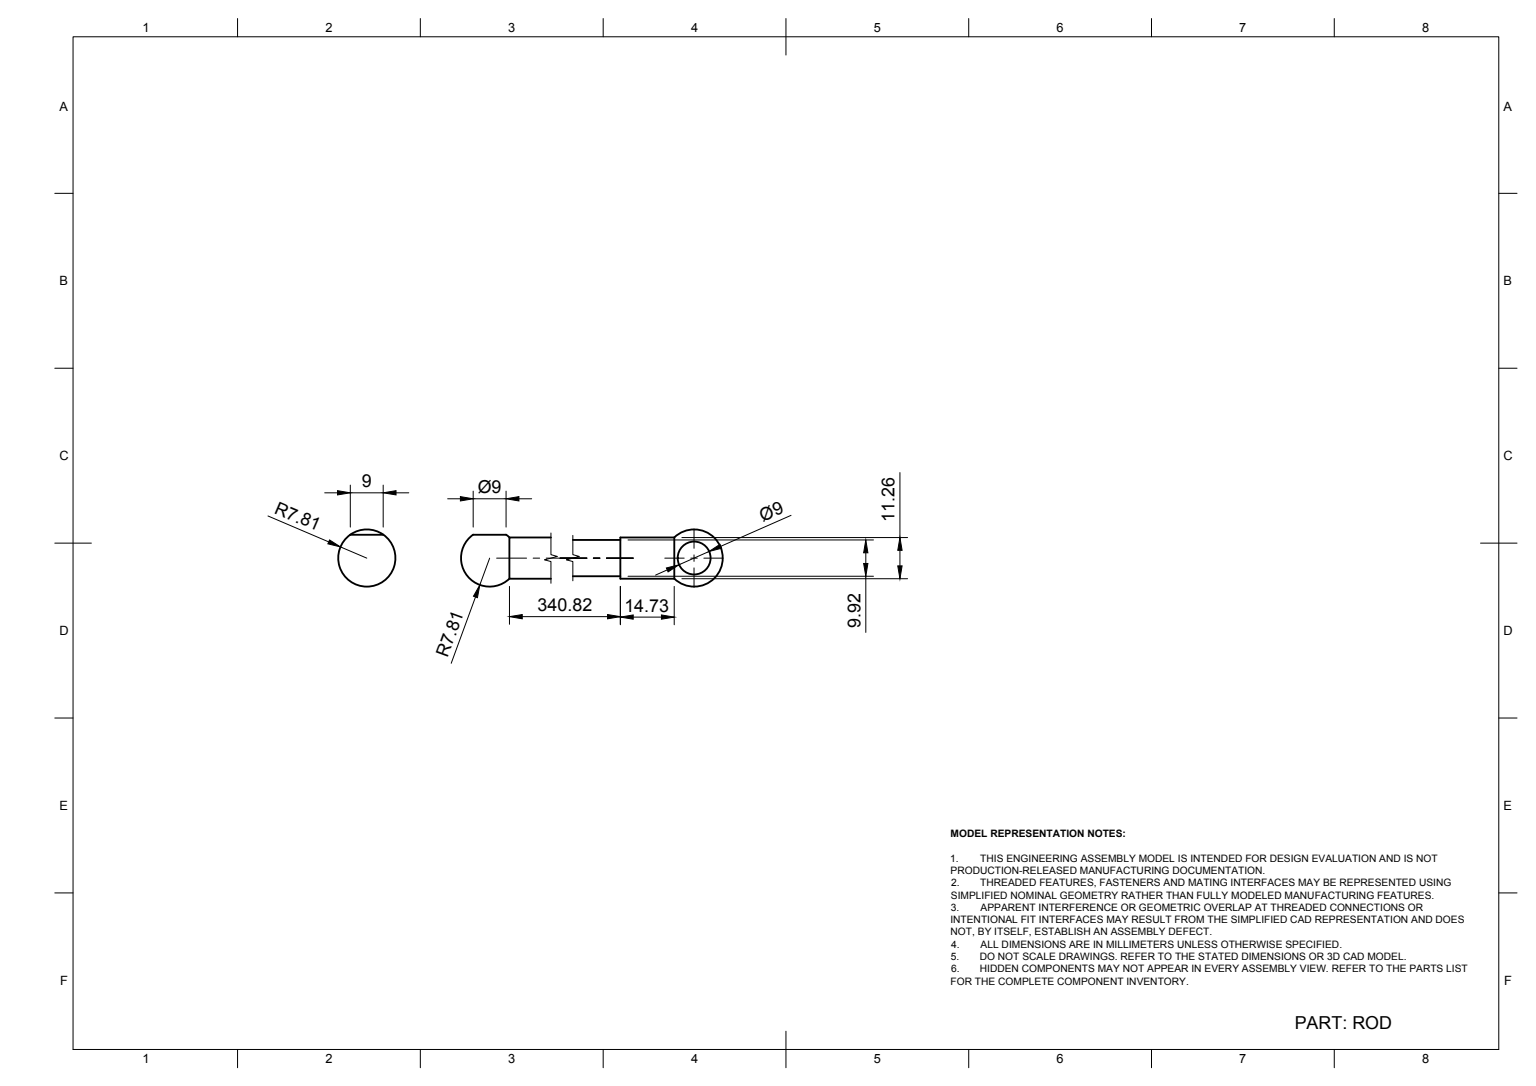
ISO-10303-21;
HEADER;
/* Generated by software containing ST-Developer
 * from STEP Tools, Inc. (www.steptools.com) 
 */

FILE_DESCRIPTION(
/* description */ (''),
/* implementation_level */ '2;1');

FILE_NAME(
/* name */ 'Rod.step',
/* time_stamp */ '2026-10-04T16:49:01-07:00',
/* author */ (''),
/* organization */ (''),
/* preprocessor_version */ 'ST-DEVELOPER v20.2',
/* originating_system */ 'Autodesk Translation Framework v15.15.0.0',
/* authorisation */ '');

FILE_SCHEMA (('AUTOMOTIVE_DESIGN { 1 0 10303 214 3 1 1 }'));
ENDSEC;

DATA;
#10=MECHANICAL_DESIGN_GEOMETRIC_PRESENTATION_REPRESENTATION('',(#87,#88),#51553);
#43=SPHERICAL_SURFACE('',#4646,7.81234603703673);
#44=SPHERICAL_SURFACE('',#4651,7.81234603703673);
#71=SHAPE_REPRESENTATION_RELATIONSHIP('SRR','None',#51592,#79);
#79=ADVANCED_BREP_SHAPE_REPRESENTATION('',(#96,#97),#51552);
#87=STYLED_ITEM('',(#51634),#96);
#88=STYLED_ITEM('',(#51634),#97);
#96=MANIFOLD_SOLID_BREP('Body1',#4266);
#97=MANIFOLD_SOLID_BREP('Body2',#4267);
#116=FACE_BOUND('',#579,.T.);
#117=FACE_BOUND('',#583,.T.);
#118=FACE_BOUND('',#586,.T.);
#119=FACE_BOUND('',#591,.T.);
#175=PLANE('',#4632);
#176=PLANE('',#4637);
#177=PLANE('',#4639);
#178=PLANE('',#4658);
#179=PLANE('',#4661);
#180=PLANE('',#4662);
#362=FACE_OUTER_BOUND('',#575,.T.);
#363=FACE_OUTER_BOUND('',#576,.T.);
#364=FACE_OUTER_BOUND('',#577,.T.);
#365=FACE_OUTER_BOUND('',#578,.T.);
#366=FACE_OUTER_BOUND('',#580,.T.);
#367=FACE_OUTER_BOUND('',#581,.T.);
#368=FACE_OUTER_BOUND('',#582,.T.);
#369=FACE_OUTER_BOUND('',#584,.T.);
#370=FACE_OUTER_BOUND('',#585,.T.);
#371=FACE_OUTER_BOUND('',#587,.T.);
#372=FACE_OUTER_BOUND('',#588,.T.);
#373=FACE_OUTER_BOUND('',#589,.T.);
#374=FACE_OUTER_BOUND('',#590,.T.);
#375=FACE_OUTER_BOUND('',#592,.T.);
#575=EDGE_LOOP('',(#3895,#3896,#3897,#3898,#3899));
#576=EDGE_LOOP('',(#3900,#3901,#3902,#3903,#3904,#3905,#3906));
#577=EDGE_LOOP('',(#3907,#3908));
#578=EDGE_LOOP('',(#3909));
#579=EDGE_LOOP('',(#3910));
#580=EDGE_LOOP('',(#3911,#3912,#3913,#3914,#3915,#3916,#3917,#3918));
#581=EDGE_LOOP('',(#3919,#3920,#3921,#3922,#3923));
#582=EDGE_LOOP('',(#3924,#3925,#3926,#3927));
#583=EDGE_LOOP('',(#3928));
#584=EDGE_LOOP('',(#3929,#3930,#3931,#3932));
#585=EDGE_LOOP('',(#3933,#3934,#3935,#3936));
#586=EDGE_LOOP('',(#3937));
#587=EDGE_LOOP('',(#3938,#3939,#3940,#3941,#3942));
#588=EDGE_LOOP('',(#3943));
#589=EDGE_LOOP('',(#3944,#3945,#3946,#3947));
#590=EDGE_LOOP('',(#3948));
#591=EDGE_LOOP('',(#3949));
#592=EDGE_LOOP('',(#3950));
#694=CIRCLE('',#4633,5.);
#695=CIRCLE('',#4634,5.);
#696=CIRCLE('',#4636,5.);
#697=CIRCLE('',#4638,4.49999999999996);
#698=CIRCLE('',#4640,5.62967641351579);
#699=CIRCLE('',#4642,4.49999999999996);
#700=CIRCLE('',#4644,5.62967641351579);
#701=CIRCLE('',#4645,5.62967641351579);
#702=CIRCLE('',#4647,7.81234603703673);
#703=CIRCLE('',#4649,4.9623029756639);
#704=CIRCLE('',#4650,4.9623029756639);
#705=CIRCLE('',#4652,5.62967641351579);
#706=CIRCLE('',#4653,5.62967641351579);
#707=CIRCLE('',#4654,7.81234603703673);
#708=CIRCLE('',#4655,4.49999999999996);
#709=CIRCLE('',#4657,5.62967641351579);
#710=CIRCLE('',#4659,4.49999999999996);
#930=LINE('',#51453,#1158);
#931=LINE('',#51459,#1159);
#932=LINE('',#51460,#1160);
#933=LINE('',#51464,#1161);
#934=LINE('',#51490,#1162);
#935=LINE('',#51493,#1163);
#936=LINE('',#51504,#1164);
#937=LINE('',#51517,#1165);
#938=LINE('',#51523,#1166);
#1158=VECTOR('',#5442,10.);
#1159=VECTOR('',#5447,10.);
#1160=VECTOR('',#5448,10.);
#1161=VECTOR('',#5453,5.);
#1162=VECTOR('',#5466,4.49999999999996);
#1163=VECTOR('',#5469,5.62967641351579);
#1164=VECTOR('',#5482,4.9623029756639);
#1165=VECTOR('',#5497,5.62967641351579);
#1166=VECTOR('',#5506,4.49999999999996);
#1480=B_SPLINE_CURVE_WITH_KNOTS('',3,(#51466,#51467,#51468,#51469,#51470,
#51471,#51472,#51473),.UNSPECIFIED.,.F.,.F.,(4,2,2,4),(2.26932848662342,
2.45137478361407,2.63342108060473,2.80969614393453),.UNSPECIFIED.);
#1481=B_SPLINE_CURVE_WITH_KNOTS('',3,(#51474,#51475,#51476,#51477,#51478,
#51479,#51480,#51481),.UNSPECIFIED.,.F.,.F.,(4,2,2,4),(1.72896082931231,
1.90523589264212,2.08728218963277,2.26932848662342),.UNSPECIFIED.);
#1948=VERTEX_POINT('',#51451);
#1949=VERTEX_POINT('',#51452);
#1950=VERTEX_POINT('',#51454);
#1951=VERTEX_POINT('',#51456);
#1952=VERTEX_POINT('',#51458);
#1953=VERTEX_POINT('',#51462);
#1954=VERTEX_POINT('',#51465);
#1955=VERTEX_POINT('',#51485);
#1956=VERTEX_POINT('',#51488);
#1957=VERTEX_POINT('',#51492);
#1958=VERTEX_POINT('',#51494);
#1959=VERTEX_POINT('',#51498);
#1960=VERTEX_POINT('',#51501);
#1961=VERTEX_POINT('',#51503);
#1962=VERTEX_POINT('',#51507);
#1963=VERTEX_POINT('',#51508);
#1964=VERTEX_POINT('',#51511);
#1965=VERTEX_POINT('',#51513);
#1966=VERTEX_POINT('',#51516);
#1967=VERTEX_POINT('',#51520);
#2601=EDGE_CURVE('',#1948,#1949,#930,.T.);
#2602=EDGE_CURVE('',#1950,#1948,#694,.T.);
#2603=EDGE_CURVE('',#1951,#1950,#695,.T.);
#2604=EDGE_CURVE('',#1952,#1951,#931,.T.);
#2605=EDGE_CURVE('',#1949,#1952,#932,.T.);
#2606=EDGE_CURVE('',#1953,#1953,#696,.T.);
#2607=EDGE_CURVE('',#1953,#1950,#933,.T.);
#2608=EDGE_CURVE('',#1954,#1948,#1480,.T.);
#2609=EDGE_CURVE('',#1951,#1954,#1481,.T.);
#2610=EDGE_CURVE('',#1952,#1949,#697,.T.);
#2611=EDGE_CURVE('',#1955,#1955,#698,.T.);
#2612=EDGE_CURVE('',#1956,#1956,#699,.T.);
#2613=EDGE_CURVE('',#1956,#1954,#934,.T.);
#2614=EDGE_CURVE('',#1955,#1957,#935,.T.);
#2615=EDGE_CURVE('',#1957,#1958,#700,.T.);
#2616=EDGE_CURVE('',#1958,#1957,#701,.T.);
#2617=EDGE_CURVE('',#1959,#1958,#702,.T.);
#2618=EDGE_CURVE('',#1960,#1960,#703,.T.);
#2619=EDGE_CURVE('',#1960,#1961,#936,.T.);
#2620=EDGE_CURVE('',#1961,#1961,#704,.T.);
#2621=EDGE_CURVE('',#1962,#1963,#705,.T.);
#2622=EDGE_CURVE('',#1963,#1962,#706,.T.);
#2623=EDGE_CURVE('',#1964,#1962,#707,.T.);
#2624=EDGE_CURVE('',#1965,#1965,#708,.T.);
#2625=EDGE_CURVE('',#1963,#1966,#937,.T.);
#2626=EDGE_CURVE('',#1966,#1966,#709,.T.);
#2627=EDGE_CURVE('',#1967,#1967,#710,.T.);
#2628=EDGE_CURVE('',#1967,#1965,#938,.T.);
#3895=ORIENTED_EDGE('',*,*,#2601,.F.);
#3896=ORIENTED_EDGE('',*,*,#2602,.F.);
#3897=ORIENTED_EDGE('',*,*,#2603,.F.);
#3898=ORIENTED_EDGE('',*,*,#2604,.F.);
#3899=ORIENTED_EDGE('',*,*,#2605,.F.);
#3900=ORIENTED_EDGE('',*,*,#2606,.F.);
#3901=ORIENTED_EDGE('',*,*,#2607,.T.);
#3902=ORIENTED_EDGE('',*,*,#2602,.T.);
#3903=ORIENTED_EDGE('',*,*,#2608,.F.);
#3904=ORIENTED_EDGE('',*,*,#2609,.F.);
#3905=ORIENTED_EDGE('',*,*,#2603,.T.);
#3906=ORIENTED_EDGE('',*,*,#2607,.F.);
#3907=ORIENTED_EDGE('',*,*,#2605,.T.);
#3908=ORIENTED_EDGE('',*,*,#2610,.T.);
#3909=ORIENTED_EDGE('',*,*,#2611,.T.);
#3910=ORIENTED_EDGE('',*,*,#2606,.T.);
#3911=ORIENTED_EDGE('',*,*,#2612,.T.);
#3912=ORIENTED_EDGE('',*,*,#2613,.T.);
#3913=ORIENTED_EDGE('',*,*,#2608,.T.);
#3914=ORIENTED_EDGE('',*,*,#2601,.T.);
#3915=ORIENTED_EDGE('',*,*,#2610,.F.);
#3916=ORIENTED_EDGE('',*,*,#2604,.T.);
#3917=ORIENTED_EDGE('',*,*,#2609,.T.);
#3918=ORIENTED_EDGE('',*,*,#2613,.F.);
#3919=ORIENTED_EDGE('',*,*,#2611,.F.);
#3920=ORIENTED_EDGE('',*,*,#2614,.T.);
#3921=ORIENTED_EDGE('',*,*,#2615,.T.);
#3922=ORIENTED_EDGE('',*,*,#2616,.T.);
#3923=ORIENTED_EDGE('',*,*,#2614,.F.);
#3924=ORIENTED_EDGE('',*,*,#2616,.F.);
#3925=ORIENTED_EDGE('',*,*,#2617,.F.);
#3926=ORIENTED_EDGE('',*,*,#2617,.T.);
#3927=ORIENTED_EDGE('',*,*,#2615,.F.);
#3928=ORIENTED_EDGE('',*,*,#2612,.F.);
#3929=ORIENTED_EDGE('',*,*,#2618,.T.);
#3930=ORIENTED_EDGE('',*,*,#2619,.T.);
#3931=ORIENTED_EDGE('',*,*,#2620,.T.);
#3932=ORIENTED_EDGE('',*,*,#2619,.F.);
#3933=ORIENTED_EDGE('',*,*,#2621,.T.);
#3934=ORIENTED_EDGE('',*,*,#2622,.T.);
#3935=ORIENTED_EDGE('',*,*,#2623,.F.);
#3936=ORIENTED_EDGE('',*,*,#2623,.T.);
#3937=ORIENTED_EDGE('',*,*,#2624,.T.);
#3938=ORIENTED_EDGE('',*,*,#2621,.F.);
#3939=ORIENTED_EDGE('',*,*,#2622,.F.);
#3940=ORIENTED_EDGE('',*,*,#2625,.T.);
#3941=ORIENTED_EDGE('',*,*,#2626,.T.);
#3942=ORIENTED_EDGE('',*,*,#2625,.F.);
#3943=ORIENTED_EDGE('',*,*,#2627,.F.);
#3944=ORIENTED_EDGE('',*,*,#2627,.T.);
#3945=ORIENTED_EDGE('',*,*,#2628,.T.);
#3946=ORIENTED_EDGE('',*,*,#2624,.F.);
#3947=ORIENTED_EDGE('',*,*,#2628,.F.);
#3948=ORIENTED_EDGE('',*,*,#2626,.F.);
#3949=ORIENTED_EDGE('',*,*,#2618,.F.);
#3950=ORIENTED_EDGE('',*,*,#2620,.F.);
#4058=CYLINDRICAL_SURFACE('',#4635,5.);
#4059=CYLINDRICAL_SURFACE('',#4641,4.49999999999996);
#4060=CYLINDRICAL_SURFACE('',#4643,5.62967641351579);
#4061=CYLINDRICAL_SURFACE('',#4648,4.9623029756639);
#4062=CYLINDRICAL_SURFACE('',#4656,5.62967641351579);
#4063=CYLINDRICAL_SURFACE('',#4660,4.49999999999996);
#4245=ADVANCED_FACE('',(#362),#175,.T.);
#4246=ADVANCED_FACE('',(#363),#4058,.F.);
#4247=ADVANCED_FACE('',(#364),#176,.T.);
#4248=ADVANCED_FACE('',(#365,#116),#177,.F.);
#4249=ADVANCED_FACE('',(#366),#4059,.F.);
#4250=ADVANCED_FACE('',(#367),#4060,.T.);
#4251=ADVANCED_FACE('',(#368,#117),#43,.T.);
#4252=ADVANCED_FACE('',(#369),#4061,.T.);
#4253=ADVANCED_FACE('',(#370,#118),#44,.T.);
#4254=ADVANCED_FACE('',(#371),#4062,.T.);
#4255=ADVANCED_FACE('',(#372),#178,.F.);
#4256=ADVANCED_FACE('',(#373),#4063,.F.);
#4257=ADVANCED_FACE('',(#374,#119),#179,.T.);
#4258=ADVANCED_FACE('',(#375),#180,.F.);
#4266=CLOSED_SHELL('',(#4245,#4246,#4247,#4248,#4249,#4250,#4251));
#4267=CLOSED_SHELL('',(#4252,#4253,#4254,#4255,#4256,#4257,#4258));
#4631=AXIS2_PLACEMENT_3D('',#51449,#5438,#5439);
#4632=AXIS2_PLACEMENT_3D('',#51450,#5440,#5441);
#4633=AXIS2_PLACEMENT_3D('',#51455,#5443,#5444);
#4634=AXIS2_PLACEMENT_3D('',#51457,#5445,#5446);
#4635=AXIS2_PLACEMENT_3D('',#51461,#5449,#5450);
#4636=AXIS2_PLACEMENT_3D('',#51463,#5451,#5452);
#4637=AXIS2_PLACEMENT_3D('',#51482,#5454,#5455);
#4638=AXIS2_PLACEMENT_3D('',#51483,#5456,#5457);
#4639=AXIS2_PLACEMENT_3D('',#51484,#5458,#5459);
#4640=AXIS2_PLACEMENT_3D('',#51486,#5460,#5461);
#4641=AXIS2_PLACEMENT_3D('',#51487,#5462,#5463);
#4642=AXIS2_PLACEMENT_3D('',#51489,#5464,#5465);
#4643=AXIS2_PLACEMENT_3D('',#51491,#5467,#5468);
#4644=AXIS2_PLACEMENT_3D('',#51495,#5470,#5471);
#4645=AXIS2_PLACEMENT_3D('',#51496,#5472,#5473);
#4646=AXIS2_PLACEMENT_3D('',#51497,#5474,#5475);
#4647=AXIS2_PLACEMENT_3D('',#51499,#5476,#5477);
#4648=AXIS2_PLACEMENT_3D('',#51500,#5478,#5479);
#4649=AXIS2_PLACEMENT_3D('',#51502,#5480,#5481);
#4650=AXIS2_PLACEMENT_3D('',#51505,#5483,#5484);
#4651=AXIS2_PLACEMENT_3D('',#51506,#5485,#5486);
#4652=AXIS2_PLACEMENT_3D('',#51509,#5487,#5488);
#4653=AXIS2_PLACEMENT_3D('',#51510,#5489,#5490);
#4654=AXIS2_PLACEMENT_3D('',#51512,#5491,#5492);
#4655=AXIS2_PLACEMENT_3D('',#51514,#5493,#5494);
#4656=AXIS2_PLACEMENT_3D('',#51515,#5495,#5496);
#4657=AXIS2_PLACEMENT_3D('',#51518,#5498,#5499);
#4658=AXIS2_PLACEMENT_3D('',#51519,#5500,#5501);
#4659=AXIS2_PLACEMENT_3D('',#51521,#5502,#5503);
#4660=AXIS2_PLACEMENT_3D('',#51522,#5504,#5505);
#4661=AXIS2_PLACEMENT_3D('',#51524,#5507,#5508);
#4662=AXIS2_PLACEMENT_3D('',#51525,#5509,#5510);
#5438=DIRECTION('axis',(0.,0.,1.));
#5439=DIRECTION('refdir',(1.,0.,0.));
#5440=DIRECTION('center_axis',(1.,0.,0.));
#5441=DIRECTION('ref_axis',(0.,1.,0.));
#5442=DIRECTION('',(0.,-2.22044604925031E-16,-1.));
#5443=DIRECTION('center_axis',(-1.,0.,0.));
#5444=DIRECTION('ref_axis',(0.,1.,0.));
#5445=DIRECTION('center_axis',(-1.,0.,0.));
#5446=DIRECTION('ref_axis',(0.,1.,0.));
#5447=DIRECTION('',(0.,2.22044604925031E-16,1.));
#5448=DIRECTION('',(0.,1.,-2.22044604925031E-16));
#5449=DIRECTION('center_axis',(-1.,0.,0.));
#5450=DIRECTION('ref_axis',(0.,1.,0.));
#5451=DIRECTION('center_axis',(-1.,0.,0.));
#5452=DIRECTION('ref_axis',(0.,1.,0.));
#5453=DIRECTION('',(-1.,0.,0.));
#5454=DIRECTION('center_axis',(0.,2.22044604925031E-16,1.));
#5455=DIRECTION('ref_axis',(-1.,0.,0.));
#5456=DIRECTION('center_axis',(0.,2.22044604925031E-16,1.));
#5457=DIRECTION('ref_axis',(-1.,0.,0.));
#5458=DIRECTION('center_axis',(-1.,0.,0.));
#5459=DIRECTION('ref_axis',(0.,1.,-2.22044604925031E-16));
#5460=DIRECTION('center_axis',(1.,0.,0.));
#5461=DIRECTION('ref_axis',(0.,-1.,2.22044604925031E-16));
#5462=DIRECTION('center_axis',(0.,-2.22044604925031E-16,-1.));
#5463=DIRECTION('ref_axis',(-1.,0.,0.));
#5464=DIRECTION('center_axis',(0.,2.22044604925031E-16,1.));
#5465=DIRECTION('ref_axis',(-1.,0.,0.));
#5466=DIRECTION('',(0.,-2.22044604925031E-16,-1.));
#5467=DIRECTION('center_axis',(1.,0.,0.));
#5468=DIRECTION('ref_axis',(0.,-1.,2.22044604925031E-16));
#5469=DIRECTION('',(-1.,0.,0.));
#5470=DIRECTION('center_axis',(1.,0.,0.));
#5471=DIRECTION('ref_axis',(0.,-1.,2.22044604925031E-16));
#5472=DIRECTION('center_axis',(1.,0.,0.));
#5473=DIRECTION('ref_axis',(0.,-1.,2.22044604925031E-16));
#5474=DIRECTION('center_axis',(-1.,2.71926214689378E-32,1.22464679914735E-16));
#5475=DIRECTION('ref_axis',(1.1368907822176E-16,2.22044604925031E-16,1.));
#5476=DIRECTION('center_axis',(7.49879891330929E-33,-1.,3.44509284839766E-16));
#5477=DIRECTION('ref_axis',(-7.10556738886E-17,-3.44509284839766E-16,-1.));
#5478=DIRECTION('center_axis',(1.,0.,0.));
#5479=DIRECTION('ref_axis',(0.,0.,-1.));
#5480=DIRECTION('center_axis',(-1.,0.,0.));
#5481=DIRECTION('ref_axis',(0.,0.,-1.));
#5482=DIRECTION('',(-1.,0.,0.));
#5483=DIRECTION('center_axis',(1.,0.,0.));
#5484=DIRECTION('ref_axis',(0.,0.,-1.));
#5485=DIRECTION('center_axis',(1.,-1.22464679914736E-16,0.));
#5486=DIRECTION('ref_axis',(0.,-1.,0.));
#5487=DIRECTION('center_axis',(1.,0.,0.));
#5488=DIRECTION('ref_axis',(0.,0.,-1.));
#5489=DIRECTION('center_axis',(1.,0.,0.));
#5490=DIRECTION('ref_axis',(0.,0.,-1.));
#5491=DIRECTION('center_axis',(-7.4987989133093E-33,-1.22464679914735E-16,
1.));
#5492=DIRECTION('ref_axis',(0.,1.,1.22464679914735E-16));
#5493=DIRECTION('center_axis',(0.,1.,0.));
#5494=DIRECTION('ref_axis',(1.,0.,0.));
#5495=DIRECTION('center_axis',(1.,0.,0.));
#5496=DIRECTION('ref_axis',(0.,0.,-1.));
#5497=DIRECTION('',(-1.,0.,0.));
#5498=DIRECTION('center_axis',(1.,0.,0.));
#5499=DIRECTION('ref_axis',(0.,0.,-1.));
#5500=DIRECTION('center_axis',(0.,1.,0.));
#5501=DIRECTION('ref_axis',(1.,0.,0.));
#5502=DIRECTION('center_axis',(0.,1.,0.));
#5503=DIRECTION('ref_axis',(1.,0.,0.));
#5504=DIRECTION('center_axis',(0.,-1.,0.));
#5505=DIRECTION('ref_axis',(1.,0.,0.));
#5506=DIRECTION('',(0.,-1.,0.));
#5507=DIRECTION('center_axis',(-1.,0.,0.));
#5508=DIRECTION('ref_axis',(0.,0.,1.));
#5509=DIRECTION('center_axis',(1.,0.,0.));
#5510=DIRECTION('ref_axis',(0.,1.,0.));
#51449=CARTESIAN_POINT('',(0.,0.,0.));
#51450=CARTESIAN_POINT('Origin',(6.37917532067789,0.,0.));
#51451=CARTESIAN_POINT('',(6.37917532067789,-4.06856249956639,2.90633776205073));
#51452=CARTESIAN_POINT('',(6.37917532067789,-4.06856249956639,9.03402352829016E-16));
#51453=CARTESIAN_POINT('',(6.37917532067789,-4.06856249956639,9.03402352829016E-16));
#51454=CARTESIAN_POINT('',(6.37917532067789,-5.,6.12323399573677E-16));
#51455=CARTESIAN_POINT('Origin',(6.37917532067789,0.,0.));
#51456=CARTESIAN_POINT('',(6.37917532067789,4.06856249956639,2.90633776205073));
#51457=CARTESIAN_POINT('Origin',(6.37917532067789,0.,0.));
#51458=CARTESIAN_POINT('',(6.37917532067789,4.06856249956639,-9.03402352829016E-16));
#51459=CARTESIAN_POINT('',(6.37917532067789,4.06856249956639,-9.03402352829016E-16));
#51460=CARTESIAN_POINT('',(6.37917532067789,0.,0.));
#51461=CARTESIAN_POINT('Origin',(206.833344075386,0.,0.));
#51462=CARTESIAN_POINT('',(24.6022815711059,-5.,6.12323399573677E-16));
#51463=CARTESIAN_POINT('Origin',(24.6022815711059,0.,0.));
#51464=CARTESIAN_POINT('',(206.833344075386,-5.,6.12323399573677E-16));
#51465=CARTESIAN_POINT('',(8.95646910621821,8.6937196433654E-16,5.));
#51466=CARTESIAN_POINT('Ctrl Pts',(8.95646910621821,1.17961196366423E-15,
5.));
#51467=CARTESIAN_POINT('Ctrl Pts',(8.95646910621821,-0.606820989968836,
5.));
#51468=CARTESIAN_POINT('Ctrl Pts',(8.82673713165736,-1.22898791230303,4.88231525391355));
#51469=CARTESIAN_POINT('Ctrl Pts',(8.35235281675177,-2.33060974443834,4.46269756160066));
#51470=CARTESIAN_POINT('Ctrl Pts',(8.00907805487115,-2.81135208202597,4.16259123013233));
#51471=CARTESIAN_POINT('Ctrl Pts',(7.27957085481457,-3.54085928208256,3.56072689165552));
#51472=CARTESIAN_POINT('Ctrl Pts',(6.8497028394201,-3.84620234546864,3.21761823198537));
#51473=CARTESIAN_POINT('Ctrl Pts',(6.37917532067789,-4.06856249956639,2.90633776205073));
#51474=CARTESIAN_POINT('Ctrl Pts',(6.37917532067789,4.06856249956639,2.90633776205073));
#51475=CARTESIAN_POINT('Ctrl Pts',(6.84970283942009,3.84620234546864,3.21761823198536));
#51476=CARTESIAN_POINT('Ctrl Pts',(7.27957085481456,3.54085928208256,3.56072689165552));
#51477=CARTESIAN_POINT('Ctrl Pts',(8.00907805487115,2.81135208202597,4.16259123013233));
#51478=CARTESIAN_POINT('Ctrl Pts',(8.35235281675177,2.33060974443835,4.46269756160066));
#51479=CARTESIAN_POINT('Ctrl Pts',(8.82673713165736,1.22898791230303,4.88231525391354));
#51480=CARTESIAN_POINT('Ctrl Pts',(8.95646910621821,0.60682098996884,5.));
#51481=CARTESIAN_POINT('Ctrl Pts',(8.95646910621821,8.32667268468867E-16,
5.));
#51482=CARTESIAN_POINT('Origin',(4.45646910621825,0.,0.));
#51483=CARTESIAN_POINT('Origin',(4.45646910621825,0.,0.));
#51484=CARTESIAN_POINT('Origin',(24.6022815711059,-5.62967641351579,1.25003927509488E-15));
#51485=CARTESIAN_POINT('',(24.6022815711059,5.62967641351579,-5.60602755090134E-16));
#51486=CARTESIAN_POINT('Origin',(24.6022815711059,0.,0.));
#51487=CARTESIAN_POINT('Origin',(4.45646910621825,0.,0.));
#51488=CARTESIAN_POINT('',(8.95646910621821,1.96909841056726E-15,6.38613737735135));
#51489=CARTESIAN_POINT('Origin',(4.45646910621825,1.41800735095096E-15,
6.38613737735135));
#51490=CARTESIAN_POINT('',(8.95646910621821,-5.51091059616304E-16,1.22366796610219E-31));
#51491=CARTESIAN_POINT('Origin',(17.2376725011568,0.,0.));
#51492=CARTESIAN_POINT('',(9.87306343120764,5.62967641351579,-5.60602755090133E-16));
#51493=CARTESIAN_POINT('',(17.2376725011568,5.62967641351579,-5.60602755090133E-16));
#51494=CARTESIAN_POINT('',(9.87306343120764,-5.60602755090134E-16,-5.62967641351579));
#51495=CARTESIAN_POINT('Origin',(9.87306343120764,0.,0.));
#51496=CARTESIAN_POINT('Origin',(9.87306343120764,0.,0.));
#51497=CARTESIAN_POINT('Origin',(4.45646910621825,0.,0.));
#51498=CARTESIAN_POINT('',(-3.35587693081848,-3.21444381174749E-32,7.67432839081512E-17));
#51499=CARTESIAN_POINT('Origin',(4.45646910621825,0.,0.));
#51500=CARTESIAN_POINT('Origin',(187.645393479721,0.,0.));
#51501=CARTESIAN_POINT('',(350.688505388337,6.07706845554618E-16,4.9623029756639));
#51502=CARTESIAN_POINT('Origin',(350.688505388337,0.,0.));
#51503=CARTESIAN_POINT('',(206.833344075386,-6.07706845554618E-16,4.9623029756639));
#51504=CARTESIAN_POINT('',(187.645393479721,-6.07706845554618E-16,4.9623029756639));
#51505=CARTESIAN_POINT('Origin',(206.833344075386,0.,0.));
#51506=CARTESIAN_POINT('Origin',(370.834317853224,0.,0.));
#51507=CARTESIAN_POINT('',(365.417723528235,5.62967641351579,6.89436520004747E-16));
#51508=CARTESIAN_POINT('',(365.417723528235,-6.89436520004746E-16,5.62967641351579));
#51509=CARTESIAN_POINT('Origin',(365.417723528235,0.,0.));
#51510=CARTESIAN_POINT('Origin',(365.417723528235,0.,0.));
#51511=CARTESIAN_POINT('',(378.646663890261,4.78368228404427E-16,1.17166423945854E-31));
#51512=CARTESIAN_POINT('Origin',(370.834317853224,0.,0.));
#51513=CARTESIAN_POINT('',(366.334317853224,-6.38613737735135,5.51091059616304E-16));
#51514=CARTESIAN_POINT('Origin',(370.834317853224,-6.38613737735135,0.));
#51515=CARTESIAN_POINT('Origin',(358.053114458286,0.,0.));
#51516=CARTESIAN_POINT('',(350.688505388337,-6.89436520004747E-16,5.62967641351579));
#51517=CARTESIAN_POINT('',(358.053114458286,-6.89436520004746E-16,5.62967641351579));
#51518=CARTESIAN_POINT('Origin',(350.688505388337,0.,0.));
#51519=CARTESIAN_POINT('Origin',(370.834317853224,0.,0.));
#51520=CARTESIAN_POINT('',(366.334317853224,0.,5.51091059616304E-16));
#51521=CARTESIAN_POINT('Origin',(370.834317853224,0.,0.));
#51522=CARTESIAN_POINT('Origin',(370.834317853224,0.,0.));
#51523=CARTESIAN_POINT('',(366.334317853224,0.,-5.51091059616304E-16));
#51524=CARTESIAN_POINT('Origin',(350.688505388337,0.,-5.62967641351579));
#51525=CARTESIAN_POINT('Origin',(206.833344075386,0.,0.));
#51542=UNCERTAINTY_MEASURE_WITH_UNIT(LENGTH_MEASURE(0.01),#51554,
'DISTANCE_ACCURACY_VALUE',
'Maximum model space distance between geometric entities at asserted c
onnectivities');
#51543=UNCERTAINTY_MEASURE_WITH_UNIT(LENGTH_MEASURE(0.01),#51554,
'DISTANCE_ACCURACY_VALUE',
'Maximum model space distance between geometric entities at asserted c
onnectivities');
#51552=(
GEOMETRIC_REPRESENTATION_CONTEXT(3)
GLOBAL_UNCERTAINTY_ASSIGNED_CONTEXT((#51542))
GLOBAL_UNIT_ASSIGNED_CONTEXT((#51554,#51556,#51557))
REPRESENTATION_CONTEXT('','3D')
);
#51553=(
GEOMETRIC_REPRESENTATION_CONTEXT(3)
GLOBAL_UNCERTAINTY_ASSIGNED_CONTEXT((#51543))
GLOBAL_UNIT_ASSIGNED_CONTEXT((#51554,#51556,#51557))
REPRESENTATION_CONTEXT('','3D')
);
#51554=(
LENGTH_UNIT()
NAMED_UNIT(*)
SI_UNIT(.MILLI.,.METRE.)
);
#51556=(
NAMED_UNIT(*)
PLANE_ANGLE_UNIT()
SI_UNIT($,.RADIAN.)
);
#51557=(
NAMED_UNIT(*)
SI_UNIT($,.STERADIAN.)
SOLID_ANGLE_UNIT()
);
#51566=SHAPE_DEFINITION_REPRESENTATION(#51575,#51592);
#51575=PRODUCT_DEFINITION_SHAPE('',$,#51602);
#51592=SHAPE_REPRESENTATION('',(#4631),#51552);
#51593=PRODUCT_DEFINITION_CONTEXT('part definition',#51622,'design');
#51602=PRODUCT_DEFINITION('Rod','Rod',#51611,#51593);
#51611=PRODUCT_DEFINITION_FORMATION('',$,#51632);
#51622=APPLICATION_CONTEXT(
'Core Data for Automotive Mechanical Design Process');
#51623=PRODUCT_CONTEXT('part definition',#51622,'mechanical');
#51632=PRODUCT('Rod','Rod',$,(#51623));
#51634=PRESENTATION_STYLE_ASSIGNMENT((#51637));
#51637=SURFACE_STYLE_USAGE(.BOTH.,#51640);
#51640=SURFACE_SIDE_STYLE('',(#51643));
#51643=SURFACE_STYLE_FILL_AREA(#51646);
#51646=FILL_AREA_STYLE('Opaque(203,203,203)',(#51649));
#51649=FILL_AREA_STYLE_COLOUR('Opaque(203,203,203)',#51652);
#51652=COLOUR_RGB('Opaque(203,203,203)', 0.09019608, 0.27058824, 0.51372549);
ENDSEC;
END-ISO-10303-21;
